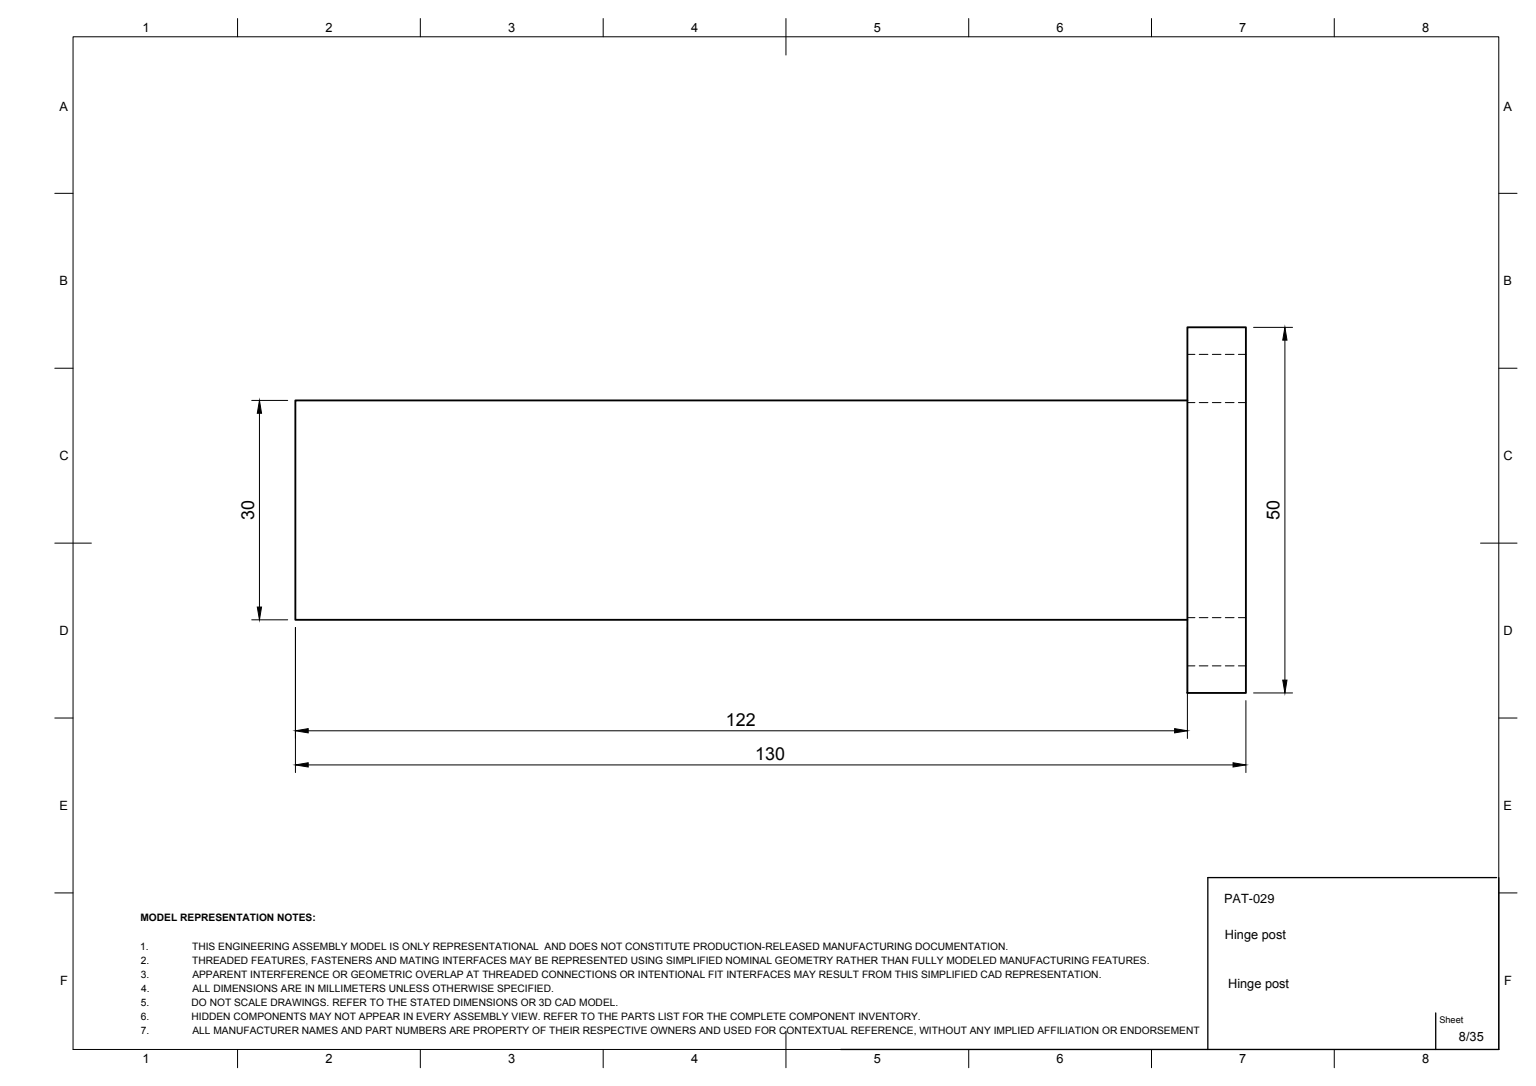
ISO-10303-21;
HEADER;
/* Generated by software containing ST-Developer
 * from STEP Tools, Inc. (www.steptools.com) 
 */

FILE_DESCRIPTION(
/* description */ ('Door-style hinge test fixture with detent'),
/* implementation_level */ '2;1');

FILE_NAME(
/* name */ 'Hinge post.step',
/* time_stamp */ '2026-10-28T03:24:57-07:00',
/* author */ (''),
/* organization */ (''),
/* preprocessor_version */ 'ST-DEVELOPER v20.2',
/* originating_system */ 'Autodesk Translation Framework v15.17.0.0',
/* authorisation */ '');

FILE_SCHEMA (('AUTOMOTIVE_DESIGN { 1 0 10303 214 3 1 1 }'));
ENDSEC;

DATA;
#10=MECHANICAL_DESIGN_GEOMETRIC_PRESENTATION_REPRESENTATION('',(#325,#326),#9813);
#263=SHAPE_REPRESENTATION_RELATIONSHIP('SRR','None',#9940,#294);
#294=ADVANCED_BREP_SHAPE_REPRESENTATION('',(#365,#366),#9783);
#325=STYLED_ITEM('',(#10169),#365);
#326=STYLED_ITEM('',(#10169),#366);
#365=MANIFOLD_SOLID_BREP('Body1',#4756);
#366=MANIFOLD_SOLID_BREP('Body2',#4757);
#407=FACE_BOUND('',#993,.T.);
#408=FACE_BOUND('',#994,.T.);
#409=FACE_BOUND('',#995,.T.);
#410=FACE_BOUND('',#996,.T.);
#411=FACE_BOUND('',#998,.T.);
#412=FACE_BOUND('',#999,.T.);
#413=FACE_BOUND('',#1000,.T.);
#414=FACE_BOUND('',#1001,.T.);
#518=PLANE('',#5174);
#519=PLANE('',#5175);
#520=PLANE('',#5176);
#521=PLANE('',#5177);
#522=PLANE('',#5178);
#523=PLANE('',#5179);
#524=PLANE('',#5192);
#525=PLANE('',#5193);
#526=PLANE('',#5194);
#527=PLANE('',#5195);
#528=PLANE('',#5196);
#529=PLANE('',#5197);
#685=FACE_OUTER_BOUND('',#978,.T.);
#686=FACE_OUTER_BOUND('',#979,.T.);
#687=FACE_OUTER_BOUND('',#980,.T.);
#688=FACE_OUTER_BOUND('',#981,.T.);
#689=FACE_OUTER_BOUND('',#982,.T.);
#690=FACE_OUTER_BOUND('',#983,.T.);
#691=FACE_OUTER_BOUND('',#984,.T.);
#692=FACE_OUTER_BOUND('',#985,.T.);
#693=FACE_OUTER_BOUND('',#986,.T.);
#694=FACE_OUTER_BOUND('',#987,.T.);
#695=FACE_OUTER_BOUND('',#988,.T.);
#696=FACE_OUTER_BOUND('',#989,.T.);
#697=FACE_OUTER_BOUND('',#990,.T.);
#698=FACE_OUTER_BOUND('',#991,.T.);
#699=FACE_OUTER_BOUND('',#992,.T.);
#700=FACE_OUTER_BOUND('',#997,.T.);
#978=EDGE_LOOP('',(#3303,#3304,#3305,#3306));
#979=EDGE_LOOP('',(#3307,#3308,#3309,#3310));
#980=EDGE_LOOP('',(#3311,#3312,#3313,#3314));
#981=EDGE_LOOP('',(#3315,#3316,#3317,#3318));
#982=EDGE_LOOP('',(#3319,#3320,#3321,#3322));
#983=EDGE_LOOP('',(#3323,#3324,#3325,#3326));
#984=EDGE_LOOP('',(#3327,#3328,#3329,#3330));
#985=EDGE_LOOP('',(#3331,#3332,#3333,#3334));
#986=EDGE_LOOP('',(#3335,#3336,#3337,#3338));
#987=EDGE_LOOP('',(#3339,#3340,#3341,#3342));
#988=EDGE_LOOP('',(#3343,#3344,#3345,#3346));
#989=EDGE_LOOP('',(#3347,#3348,#3349,#3350));
#990=EDGE_LOOP('',(#3351,#3352,#3353,#3354));
#991=EDGE_LOOP('',(#3355,#3356,#3357,#3358));
#992=EDGE_LOOP('',(#3359,#3360,#3361,#3362));
#993=EDGE_LOOP('',(#3363));
#994=EDGE_LOOP('',(#3364));
#995=EDGE_LOOP('',(#3365));
#996=EDGE_LOOP('',(#3366));
#997=EDGE_LOOP('',(#3367,#3368,#3369,#3370));
#998=EDGE_LOOP('',(#3371));
#999=EDGE_LOOP('',(#3372));
#1000=EDGE_LOOP('',(#3373));
#1001=EDGE_LOOP('',(#3374));
#1374=LINE('',#7408,#1694);
#1375=LINE('',#7410,#1695);
#1376=LINE('',#7412,#1696);
#1377=LINE('',#7413,#1697);
#1378=LINE('',#7416,#1698);
#1379=LINE('',#7418,#1699);
#1380=LINE('',#7419,#1700);
#1381=LINE('',#7422,#1701);
#1382=LINE('',#7424,#1702);
#1383=LINE('',#7425,#1703);
#1384=LINE('',#7427,#1704);
#1385=LINE('',#7428,#1705);
#1386=LINE('',#7435,#1706);
#1387=LINE('',#7441,#1707);
#1388=LINE('',#7447,#1708);
#1389=LINE('',#7453,#1709);
#1390=LINE('',#7458,#1710);
#1391=LINE('',#7460,#1711);
#1392=LINE('',#7462,#1712);
#1393=LINE('',#7463,#1713);
#1394=LINE('',#7466,#1714);
#1395=LINE('',#7468,#1715);
#1396=LINE('',#7469,#1716);
#1397=LINE('',#7472,#1717);
#1398=LINE('',#7474,#1718);
#1399=LINE('',#7475,#1719);
#1400=LINE('',#7477,#1720);
#1401=LINE('',#7478,#1721);
#1694=VECTOR('',#5865,1.);
#1695=VECTOR('',#5866,1.);
#1696=VECTOR('',#5867,1.);
#1697=VECTOR('',#5868,1.);
#1698=VECTOR('',#5871,1.);
#1699=VECTOR('',#5872,1.);
#1700=VECTOR('',#5873,1.);
#1701=VECTOR('',#5876,1.);
#1702=VECTOR('',#5877,1.);
#1703=VECTOR('',#5878,1.);
#1704=VECTOR('',#5881,1.);
#1705=VECTOR('',#5882,1.);
#1706=VECTOR('',#5891,0.33);
#1707=VECTOR('',#5898,0.33);
#1708=VECTOR('',#5905,0.33);
#1709=VECTOR('',#5912,0.33);
#1710=VECTOR('',#5917,1.);
#1711=VECTOR('',#5918,1.);
#1712=VECTOR('',#5919,1.);
#1713=VECTOR('',#5920,1.);
#1714=VECTOR('',#5923,1.);
#1715=VECTOR('',#5924,1.);
#1716=VECTOR('',#5925,1.);
#1717=VECTOR('',#5928,1.);
#1718=VECTOR('',#5929,1.);
#1719=VECTOR('',#5930,1.);
#1720=VECTOR('',#5933,1.);
#1721=VECTOR('',#5934,1.);
#1982=CIRCLE('',#5181,0.33);
#1983=CIRCLE('',#5182,0.33);
#1984=CIRCLE('',#5184,0.33);
#1985=CIRCLE('',#5185,0.33);
#1986=CIRCLE('',#5187,0.33);
#1987=CIRCLE('',#5188,0.33);
#1988=CIRCLE('',#5190,0.33);
#1989=CIRCLE('',#5191,0.33);
#2253=VERTEX_POINT('',#7406);
#2254=VERTEX_POINT('',#7407);
#2255=VERTEX_POINT('',#7409);
#2256=VERTEX_POINT('',#7411);
#2257=VERTEX_POINT('',#7415);
#2258=VERTEX_POINT('',#7417);
#2259=VERTEX_POINT('',#7421);
#2260=VERTEX_POINT('',#7423);
#2261=VERTEX_POINT('',#7432);
#2262=VERTEX_POINT('',#7434);
#2263=VERTEX_POINT('',#7438);
#2264=VERTEX_POINT('',#7440);
#2265=VERTEX_POINT('',#7444);
#2266=VERTEX_POINT('',#7446);
#2267=VERTEX_POINT('',#7450);
#2268=VERTEX_POINT('',#7452);
#2269=VERTEX_POINT('',#7456);
#2270=VERTEX_POINT('',#7457);
#2271=VERTEX_POINT('',#7459);
#2272=VERTEX_POINT('',#7461);
#2273=VERTEX_POINT('',#7465);
#2274=VERTEX_POINT('',#7467);
#2275=VERTEX_POINT('',#7471);
#2276=VERTEX_POINT('',#7473);
#2668=EDGE_CURVE('',#2253,#2254,#1374,.T.);
#2669=EDGE_CURVE('',#2254,#2255,#1375,.T.);
#2670=EDGE_CURVE('',#2256,#2255,#1376,.T.);
#2671=EDGE_CURVE('',#2253,#2256,#1377,.T.);
#2672=EDGE_CURVE('',#2257,#2253,#1378,.T.);
#2673=EDGE_CURVE('',#2258,#2256,#1379,.T.);
#2674=EDGE_CURVE('',#2257,#2258,#1380,.T.);
#2675=EDGE_CURVE('',#2259,#2257,#1381,.T.);
#2676=EDGE_CURVE('',#2260,#2258,#1382,.T.);
#2677=EDGE_CURVE('',#2259,#2260,#1383,.T.);
#2678=EDGE_CURVE('',#2254,#2259,#1384,.T.);
#2679=EDGE_CURVE('',#2255,#2260,#1385,.T.);
#2680=EDGE_CURVE('',#2261,#2261,#1982,.T.);
#2681=EDGE_CURVE('',#2261,#2262,#1386,.T.);
#2682=EDGE_CURVE('',#2262,#2262,#1983,.T.);
#2683=EDGE_CURVE('',#2263,#2263,#1984,.T.);
#2684=EDGE_CURVE('',#2263,#2264,#1387,.T.);
#2685=EDGE_CURVE('',#2264,#2264,#1985,.T.);
#2686=EDGE_CURVE('',#2265,#2265,#1986,.T.);
#2687=EDGE_CURVE('',#2265,#2266,#1388,.T.);
#2688=EDGE_CURVE('',#2266,#2266,#1987,.T.);
#2689=EDGE_CURVE('',#2267,#2267,#1988,.T.);
#2690=EDGE_CURVE('',#2267,#2268,#1389,.T.);
#2691=EDGE_CURVE('',#2268,#2268,#1989,.T.);
#2692=EDGE_CURVE('',#2269,#2270,#1390,.T.);
#2693=EDGE_CURVE('',#2270,#2271,#1391,.T.);
#2694=EDGE_CURVE('',#2272,#2271,#1392,.T.);
#2695=EDGE_CURVE('',#2269,#2272,#1393,.T.);
#2696=EDGE_CURVE('',#2273,#2269,#1394,.T.);
#2697=EDGE_CURVE('',#2274,#2272,#1395,.T.);
#2698=EDGE_CURVE('',#2273,#2274,#1396,.T.);
#2699=EDGE_CURVE('',#2275,#2273,#1397,.T.);
#2700=EDGE_CURVE('',#2276,#2274,#1398,.T.);
#2701=EDGE_CURVE('',#2275,#2276,#1399,.T.);
#2702=EDGE_CURVE('',#2270,#2275,#1400,.T.);
#2703=EDGE_CURVE('',#2271,#2276,#1401,.T.);
#3303=ORIENTED_EDGE('',*,*,#2668,.T.);
#3304=ORIENTED_EDGE('',*,*,#2669,.T.);
#3305=ORIENTED_EDGE('',*,*,#2670,.F.);
#3306=ORIENTED_EDGE('',*,*,#2671,.F.);
#3307=ORIENTED_EDGE('',*,*,#2672,.T.);
#3308=ORIENTED_EDGE('',*,*,#2671,.T.);
#3309=ORIENTED_EDGE('',*,*,#2673,.F.);
#3310=ORIENTED_EDGE('',*,*,#2674,.F.);
#3311=ORIENTED_EDGE('',*,*,#2675,.T.);
#3312=ORIENTED_EDGE('',*,*,#2674,.T.);
#3313=ORIENTED_EDGE('',*,*,#2676,.F.);
#3314=ORIENTED_EDGE('',*,*,#2677,.F.);
#3315=ORIENTED_EDGE('',*,*,#2678,.T.);
#3316=ORIENTED_EDGE('',*,*,#2677,.T.);
#3317=ORIENTED_EDGE('',*,*,#2679,.F.);
#3318=ORIENTED_EDGE('',*,*,#2669,.F.);
#3319=ORIENTED_EDGE('',*,*,#2679,.T.);
#3320=ORIENTED_EDGE('',*,*,#2676,.T.);
#3321=ORIENTED_EDGE('',*,*,#2673,.T.);
#3322=ORIENTED_EDGE('',*,*,#2670,.T.);
#3323=ORIENTED_EDGE('',*,*,#2678,.F.);
#3324=ORIENTED_EDGE('',*,*,#2668,.F.);
#3325=ORIENTED_EDGE('',*,*,#2672,.F.);
#3326=ORIENTED_EDGE('',*,*,#2675,.F.);
#3327=ORIENTED_EDGE('',*,*,#2680,.F.);
#3328=ORIENTED_EDGE('',*,*,#2681,.T.);
#3329=ORIENTED_EDGE('',*,*,#2682,.F.);
#3330=ORIENTED_EDGE('',*,*,#2681,.F.);
#3331=ORIENTED_EDGE('',*,*,#2683,.F.);
#3332=ORIENTED_EDGE('',*,*,#2684,.T.);
#3333=ORIENTED_EDGE('',*,*,#2685,.F.);
#3334=ORIENTED_EDGE('',*,*,#2684,.F.);
#3335=ORIENTED_EDGE('',*,*,#2686,.F.);
#3336=ORIENTED_EDGE('',*,*,#2687,.T.);
#3337=ORIENTED_EDGE('',*,*,#2688,.F.);
#3338=ORIENTED_EDGE('',*,*,#2687,.F.);
#3339=ORIENTED_EDGE('',*,*,#2689,.F.);
#3340=ORIENTED_EDGE('',*,*,#2690,.T.);
#3341=ORIENTED_EDGE('',*,*,#2691,.F.);
#3342=ORIENTED_EDGE('',*,*,#2690,.F.);
#3343=ORIENTED_EDGE('',*,*,#2692,.T.);
#3344=ORIENTED_EDGE('',*,*,#2693,.T.);
#3345=ORIENTED_EDGE('',*,*,#2694,.F.);
#3346=ORIENTED_EDGE('',*,*,#2695,.F.);
#3347=ORIENTED_EDGE('',*,*,#2696,.T.);
#3348=ORIENTED_EDGE('',*,*,#2695,.T.);
#3349=ORIENTED_EDGE('',*,*,#2697,.F.);
#3350=ORIENTED_EDGE('',*,*,#2698,.F.);
#3351=ORIENTED_EDGE('',*,*,#2699,.T.);
#3352=ORIENTED_EDGE('',*,*,#2698,.T.);
#3353=ORIENTED_EDGE('',*,*,#2700,.F.);
#3354=ORIENTED_EDGE('',*,*,#2701,.F.);
#3355=ORIENTED_EDGE('',*,*,#2702,.T.);
#3356=ORIENTED_EDGE('',*,*,#2701,.T.);
#3357=ORIENTED_EDGE('',*,*,#2703,.F.);
#3358=ORIENTED_EDGE('',*,*,#2693,.F.);
#3359=ORIENTED_EDGE('',*,*,#2703,.T.);
#3360=ORIENTED_EDGE('',*,*,#2700,.T.);
#3361=ORIENTED_EDGE('',*,*,#2697,.T.);
#3362=ORIENTED_EDGE('',*,*,#2694,.T.);
#3363=ORIENTED_EDGE('',*,*,#2682,.T.);
#3364=ORIENTED_EDGE('',*,*,#2685,.T.);
#3365=ORIENTED_EDGE('',*,*,#2688,.T.);
#3366=ORIENTED_EDGE('',*,*,#2691,.T.);
#3367=ORIENTED_EDGE('',*,*,#2702,.F.);
#3368=ORIENTED_EDGE('',*,*,#2692,.F.);
#3369=ORIENTED_EDGE('',*,*,#2696,.F.);
#3370=ORIENTED_EDGE('',*,*,#2699,.F.);
#3371=ORIENTED_EDGE('',*,*,#2680,.T.);
#3372=ORIENTED_EDGE('',*,*,#2683,.T.);
#3373=ORIENTED_EDGE('',*,*,#2686,.T.);
#3374=ORIENTED_EDGE('',*,*,#2689,.T.);
#4385=CYLINDRICAL_SURFACE('',#5180,0.33);
#4386=CYLINDRICAL_SURFACE('',#5183,0.33);
#4387=CYLINDRICAL_SURFACE('',#5186,0.33);
#4388=CYLINDRICAL_SURFACE('',#5189,0.33);
#4490=ADVANCED_FACE('',(#685),#518,.T.);
#4491=ADVANCED_FACE('',(#686),#519,.T.);
#4492=ADVANCED_FACE('',(#687),#520,.T.);
#4493=ADVANCED_FACE('',(#688),#521,.T.);
#4494=ADVANCED_FACE('',(#689),#522,.T.);
#4495=ADVANCED_FACE('',(#690),#523,.F.);
#4496=ADVANCED_FACE('',(#691),#4385,.F.);
#4497=ADVANCED_FACE('',(#692),#4386,.F.);
#4498=ADVANCED_FACE('',(#693),#4387,.F.);
#4499=ADVANCED_FACE('',(#694),#4388,.F.);
#4500=ADVANCED_FACE('',(#695),#524,.T.);
#4501=ADVANCED_FACE('',(#696),#525,.T.);
#4502=ADVANCED_FACE('',(#697),#526,.T.);
#4503=ADVANCED_FACE('',(#698),#527,.T.);
#4504=ADVANCED_FACE('',(#699,#407,#408,#409,#410),#528,.T.);
#4505=ADVANCED_FACE('',(#700,#411,#412,#413,#414),#529,.F.);
#4756=CLOSED_SHELL('',(#4490,#4491,#4492,#4493,#4494,#4495));
#4757=CLOSED_SHELL('',(#4496,#4497,#4498,#4499,#4500,#4501,#4502,#4503,
#4504,#4505));
#5173=AXIS2_PLACEMENT_3D('',#7404,#5861,#5862);
#5174=AXIS2_PLACEMENT_3D('',#7405,#5863,#5864);
#5175=AXIS2_PLACEMENT_3D('',#7414,#5869,#5870);
#5176=AXIS2_PLACEMENT_3D('',#7420,#5874,#5875);
#5177=AXIS2_PLACEMENT_3D('',#7426,#5879,#5880);
#5178=AXIS2_PLACEMENT_3D('',#7429,#5883,#5884);
#5179=AXIS2_PLACEMENT_3D('',#7430,#5885,#5886);
#5180=AXIS2_PLACEMENT_3D('',#7431,#5887,#5888);
#5181=AXIS2_PLACEMENT_3D('',#7433,#5889,#5890);
#5182=AXIS2_PLACEMENT_3D('',#7436,#5892,#5893);
#5183=AXIS2_PLACEMENT_3D('',#7437,#5894,#5895);
#5184=AXIS2_PLACEMENT_3D('',#7439,#5896,#5897);
#5185=AXIS2_PLACEMENT_3D('',#7442,#5899,#5900);
#5186=AXIS2_PLACEMENT_3D('',#7443,#5901,#5902);
#5187=AXIS2_PLACEMENT_3D('',#7445,#5903,#5904);
#5188=AXIS2_PLACEMENT_3D('',#7448,#5906,#5907);
#5189=AXIS2_PLACEMENT_3D('',#7449,#5908,#5909);
#5190=AXIS2_PLACEMENT_3D('',#7451,#5910,#5911);
#5191=AXIS2_PLACEMENT_3D('',#7454,#5913,#5914);
#5192=AXIS2_PLACEMENT_3D('',#7455,#5915,#5916);
#5193=AXIS2_PLACEMENT_3D('',#7464,#5921,#5922);
#5194=AXIS2_PLACEMENT_3D('',#7470,#5926,#5927);
#5195=AXIS2_PLACEMENT_3D('',#7476,#5931,#5932);
#5196=AXIS2_PLACEMENT_3D('',#7479,#5935,#5936);
#5197=AXIS2_PLACEMENT_3D('',#7480,#5937,#5938);
#5861=DIRECTION('axis',(0.,0.,1.));
#5862=DIRECTION('refdir',(1.,0.,0.));
#5863=DIRECTION('center_axis',(0.,1.,0.));
#5864=DIRECTION('ref_axis',(-1.,0.,0.));
#5865=DIRECTION('',(-1.,0.,0.));
#5866=DIRECTION('',(0.,0.,1.));
#5867=DIRECTION('',(-1.,0.,0.));
#5868=DIRECTION('',(0.,0.,1.));
#5869=DIRECTION('center_axis',(1.,0.,0.));
#5870=DIRECTION('ref_axis',(0.,1.,0.));
#5871=DIRECTION('',(0.,1.,0.));
#5872=DIRECTION('',(0.,1.,0.));
#5873=DIRECTION('',(0.,0.,1.));
#5874=DIRECTION('center_axis',(0.,-1.,0.));
#5875=DIRECTION('ref_axis',(1.,0.,0.));
#5876=DIRECTION('',(1.,0.,0.));
#5877=DIRECTION('',(1.,0.,0.));
#5878=DIRECTION('',(0.,0.,1.));
#5879=DIRECTION('center_axis',(-1.,0.,0.));
#5880=DIRECTION('ref_axis',(0.,-1.,0.));
#5881=DIRECTION('',(0.,-1.,0.));
#5882=DIRECTION('',(0.,-1.,0.));
#5883=DIRECTION('center_axis',(0.,0.,1.));
#5884=DIRECTION('ref_axis',(1.,0.,0.));
#5885=DIRECTION('center_axis',(0.,0.,1.));
#5886=DIRECTION('ref_axis',(1.,0.,0.));
#5887=DIRECTION('center_axis',(0.,0.,1.));
#5888=DIRECTION('ref_axis',(1.,0.,0.));
#5889=DIRECTION('center_axis',(0.,0.,1.));
#5890=DIRECTION('ref_axis',(1.,0.,0.));
#5891=DIRECTION('',(0.,0.,1.));
#5892=DIRECTION('center_axis',(0.,0.,-1.));
#5893=DIRECTION('ref_axis',(1.,0.,0.));
#5894=DIRECTION('center_axis',(0.,0.,1.));
#5895=DIRECTION('ref_axis',(1.,0.,0.));
#5896=DIRECTION('center_axis',(0.,0.,1.));
#5897=DIRECTION('ref_axis',(1.,0.,0.));
#5898=DIRECTION('',(0.,0.,1.));
#5899=DIRECTION('center_axis',(0.,0.,-1.));
#5900=DIRECTION('ref_axis',(1.,0.,0.));
#5901=DIRECTION('center_axis',(0.,0.,1.));
#5902=DIRECTION('ref_axis',(1.,0.,0.));
#5903=DIRECTION('center_axis',(0.,0.,1.));
#5904=DIRECTION('ref_axis',(1.,0.,0.));
#5905=DIRECTION('',(0.,0.,1.));
#5906=DIRECTION('center_axis',(0.,0.,-1.));
#5907=DIRECTION('ref_axis',(1.,0.,0.));
#5908=DIRECTION('center_axis',(0.,0.,1.));
#5909=DIRECTION('ref_axis',(1.,0.,0.));
#5910=DIRECTION('center_axis',(0.,0.,1.));
#5911=DIRECTION('ref_axis',(1.,0.,0.));
#5912=DIRECTION('',(0.,0.,1.));
#5913=DIRECTION('center_axis',(0.,0.,-1.));
#5914=DIRECTION('ref_axis',(1.,0.,0.));
#5915=DIRECTION('center_axis',(0.,1.,0.));
#5916=DIRECTION('ref_axis',(-1.,0.,0.));
#5917=DIRECTION('',(-1.,0.,0.));
#5918=DIRECTION('',(0.,0.,1.));
#5919=DIRECTION('',(-1.,0.,0.));
#5920=DIRECTION('',(0.,0.,1.));
#5921=DIRECTION('center_axis',(1.,0.,0.));
#5922=DIRECTION('ref_axis',(0.,1.,0.));
#5923=DIRECTION('',(0.,1.,0.));
#5924=DIRECTION('',(0.,1.,0.));
#5925=DIRECTION('',(0.,0.,1.));
#5926=DIRECTION('center_axis',(0.,-1.,0.));
#5927=DIRECTION('ref_axis',(1.,0.,0.));
#5928=DIRECTION('',(1.,0.,0.));
#5929=DIRECTION('',(1.,0.,0.));
#5930=DIRECTION('',(0.,0.,1.));
#5931=DIRECTION('center_axis',(-1.,0.,0.));
#5932=DIRECTION('ref_axis',(0.,-1.,0.));
#5933=DIRECTION('',(0.,-1.,0.));
#5934=DIRECTION('',(0.,-1.,0.));
#5935=DIRECTION('center_axis',(0.,0.,1.));
#5936=DIRECTION('ref_axis',(1.,0.,0.));
#5937=DIRECTION('center_axis',(0.,0.,1.));
#5938=DIRECTION('ref_axis',(1.,0.,0.));
#7404=CARTESIAN_POINT('',(0.,0.,0.));
#7405=CARTESIAN_POINT('Origin',(-3.,1.5,0.8));
#7406=CARTESIAN_POINT('',(-3.,1.5,0.8));
#7407=CARTESIAN_POINT('',(-4.5,1.5,0.8));
#7408=CARTESIAN_POINT('',(-3.,1.5,0.8));
#7409=CARTESIAN_POINT('',(-4.5,1.5,13.));
#7410=CARTESIAN_POINT('',(-4.5,1.5,0.8));
#7411=CARTESIAN_POINT('',(-3.,1.5,13.));
#7412=CARTESIAN_POINT('',(-3.,1.5,13.));
#7413=CARTESIAN_POINT('',(-3.,1.5,0.8));
#7414=CARTESIAN_POINT('Origin',(-3.,-1.5,0.8));
#7415=CARTESIAN_POINT('',(-3.,-1.5,0.8));
#7416=CARTESIAN_POINT('',(-3.,-1.5,0.8));
#7417=CARTESIAN_POINT('',(-3.,-1.5,13.));
#7418=CARTESIAN_POINT('',(-3.,-1.5,13.));
#7419=CARTESIAN_POINT('',(-3.,-1.5,0.8));
#7420=CARTESIAN_POINT('Origin',(-4.5,-1.5,0.8));
#7421=CARTESIAN_POINT('',(-4.5,-1.5,0.8));
#7422=CARTESIAN_POINT('',(-4.5,-1.5,0.8));
#7423=CARTESIAN_POINT('',(-4.5,-1.5,13.));
#7424=CARTESIAN_POINT('',(-4.5,-1.5,13.));
#7425=CARTESIAN_POINT('',(-4.5,-1.5,0.8));
#7426=CARTESIAN_POINT('Origin',(-4.5,1.5,0.8));
#7427=CARTESIAN_POINT('',(-4.5,1.5,0.8));
#7428=CARTESIAN_POINT('',(-4.5,1.5,13.));
#7429=CARTESIAN_POINT('Origin',(-3.75,0.,13.));
#7430=CARTESIAN_POINT('Origin',(-3.75,0.,0.8));
#7431=CARTESIAN_POINT('Origin',(-2.2,-1.8,-0.1));
#7432=CARTESIAN_POINT('',(-2.53,-1.8,0.));
#7433=CARTESIAN_POINT('Origin',(-2.2,-1.8,0.));
#7434=CARTESIAN_POINT('',(-2.53,-1.8,0.8));
#7435=CARTESIAN_POINT('',(-2.53,-1.8,-0.1));
#7436=CARTESIAN_POINT('Origin',(-2.2,-1.8,0.8));
#7437=CARTESIAN_POINT('Origin',(-5.3,1.8,-0.1));
#7438=CARTESIAN_POINT('',(-5.63,1.8,0.));
#7439=CARTESIAN_POINT('Origin',(-5.3,1.8,0.));
#7440=CARTESIAN_POINT('',(-5.63,1.8,0.8));
#7441=CARTESIAN_POINT('',(-5.63,1.8,-0.1));
#7442=CARTESIAN_POINT('Origin',(-5.3,1.8,0.8));
#7443=CARTESIAN_POINT('Origin',(-5.3,-1.8,-0.1));
#7444=CARTESIAN_POINT('',(-5.63,-1.8,0.));
#7445=CARTESIAN_POINT('Origin',(-5.3,-1.8,0.));
#7446=CARTESIAN_POINT('',(-5.63,-1.8,0.8));
#7447=CARTESIAN_POINT('',(-5.63,-1.8,-0.1));
#7448=CARTESIAN_POINT('Origin',(-5.3,-1.8,0.8));
#7449=CARTESIAN_POINT('Origin',(-2.2,1.8,-0.1));
#7450=CARTESIAN_POINT('',(-2.53,1.8,0.));
#7451=CARTESIAN_POINT('Origin',(-2.2,1.8,0.));
#7452=CARTESIAN_POINT('',(-2.53,1.8,0.8));
#7453=CARTESIAN_POINT('',(-2.53,1.8,-0.1));
#7454=CARTESIAN_POINT('Origin',(-2.2,1.8,0.8));
#7455=CARTESIAN_POINT('Origin',(-1.5,2.5,0.));
#7456=CARTESIAN_POINT('',(-1.5,2.5,0.));
#7457=CARTESIAN_POINT('',(-6.,2.5,0.));
#7458=CARTESIAN_POINT('',(-1.5,2.5,0.));
#7459=CARTESIAN_POINT('',(-6.,2.5,0.8));
#7460=CARTESIAN_POINT('',(-6.,2.5,0.));
#7461=CARTESIAN_POINT('',(-1.5,2.5,0.8));
#7462=CARTESIAN_POINT('',(-1.5,2.5,0.8));
#7463=CARTESIAN_POINT('',(-1.5,2.5,0.));
#7464=CARTESIAN_POINT('Origin',(-1.5,-2.5,0.));
#7465=CARTESIAN_POINT('',(-1.5,-2.5,0.));
#7466=CARTESIAN_POINT('',(-1.5,-2.5,0.));
#7467=CARTESIAN_POINT('',(-1.5,-2.5,0.8));
#7468=CARTESIAN_POINT('',(-1.5,-2.5,0.8));
#7469=CARTESIAN_POINT('',(-1.5,-2.5,0.));
#7470=CARTESIAN_POINT('Origin',(-6.,-2.5,0.));
#7471=CARTESIAN_POINT('',(-6.,-2.5,0.));
#7472=CARTESIAN_POINT('',(-6.,-2.5,0.));
#7473=CARTESIAN_POINT('',(-6.,-2.5,0.8));
#7474=CARTESIAN_POINT('',(-6.,-2.5,0.8));
#7475=CARTESIAN_POINT('',(-6.,-2.5,0.));
#7476=CARTESIAN_POINT('Origin',(-6.,2.5,0.));
#7477=CARTESIAN_POINT('',(-6.,2.5,0.));
#7478=CARTESIAN_POINT('',(-6.,2.5,0.8));
#7479=CARTESIAN_POINT('Origin',(-3.75,0.,0.8));
#7480=CARTESIAN_POINT('Origin',(-3.75,0.,0.));
#9747=UNCERTAINTY_MEASURE_WITH_UNIT(LENGTH_MEASURE(0.001),#9814,
'DISTANCE_ACCURACY_VALUE',
'Maximum model space distance between geometric entities at asserted c
onnectivities');
#9777=UNCERTAINTY_MEASURE_WITH_UNIT(LENGTH_MEASURE(0.001),#9814,
'DISTANCE_ACCURACY_VALUE',
'Maximum model space distance between geometric entities at asserted c
onnectivities');
#9783=(
GEOMETRIC_REPRESENTATION_CONTEXT(3)
GLOBAL_UNCERTAINTY_ASSIGNED_CONTEXT((#9747))
GLOBAL_UNIT_ASSIGNED_CONTEXT((#9814,#9816,#9817))
REPRESENTATION_CONTEXT('','3D')
);
#9813=(
GEOMETRIC_REPRESENTATION_CONTEXT(3)
GLOBAL_UNCERTAINTY_ASSIGNED_CONTEXT((#9777))
GLOBAL_UNIT_ASSIGNED_CONTEXT((#9814,#9816,#9817))
REPRESENTATION_CONTEXT('','3D')
);
#9814=(
LENGTH_UNIT()
NAMED_UNIT(*)
SI_UNIT(.CENTI.,.METRE.)
);
#9816=(
NAMED_UNIT(*)
PLANE_ANGLE_UNIT()
SI_UNIT($,.RADIAN.)
);
#9817=(
NAMED_UNIT(*)
SI_UNIT($,.STERADIAN.)
SOLID_ANGLE_UNIT()
);
#9823=SHAPE_DEFINITION_REPRESENTATION(#9858,#9940);
#9858=PRODUCT_DEFINITION_SHAPE('',$,#9976);
#9940=SHAPE_REPRESENTATION('',(#5173),#9783);
#9970=PRODUCT_DEFINITION_CONTEXT('part definition',#10077,'design');
#9976=PRODUCT_DEFINITION('Hinge post','Hinge post',#10011,#9970);
#10011=PRODUCT_DEFINITION_FORMATION('',$,#10084);
#10077=APPLICATION_CONTEXT(
'Core Data for Automotive Mechanical Design Process');
#10078=PRODUCT_CONTEXT('part definition',#10077,'mechanical');
#10084=PRODUCT('Hinge post','Hinge post','Hinge post',(#10078));
#10163=COLOUR_RGB('Light Blue',0.38,0.62,0.78);
#10164=FILL_AREA_STYLE_COLOUR('',#10163);
#10165=FILL_AREA_STYLE('',(#10164));
#10166=SURFACE_STYLE_FILL_AREA(#10165);
#10167=SURFACE_SIDE_STYLE('',(#10166));
#10168=SURFACE_STYLE_USAGE(.BOTH.,#10167);
#10169=PRESENTATION_STYLE_ASSIGNMENT((#10168));
ENDSEC;
END-ISO-10303-21;
